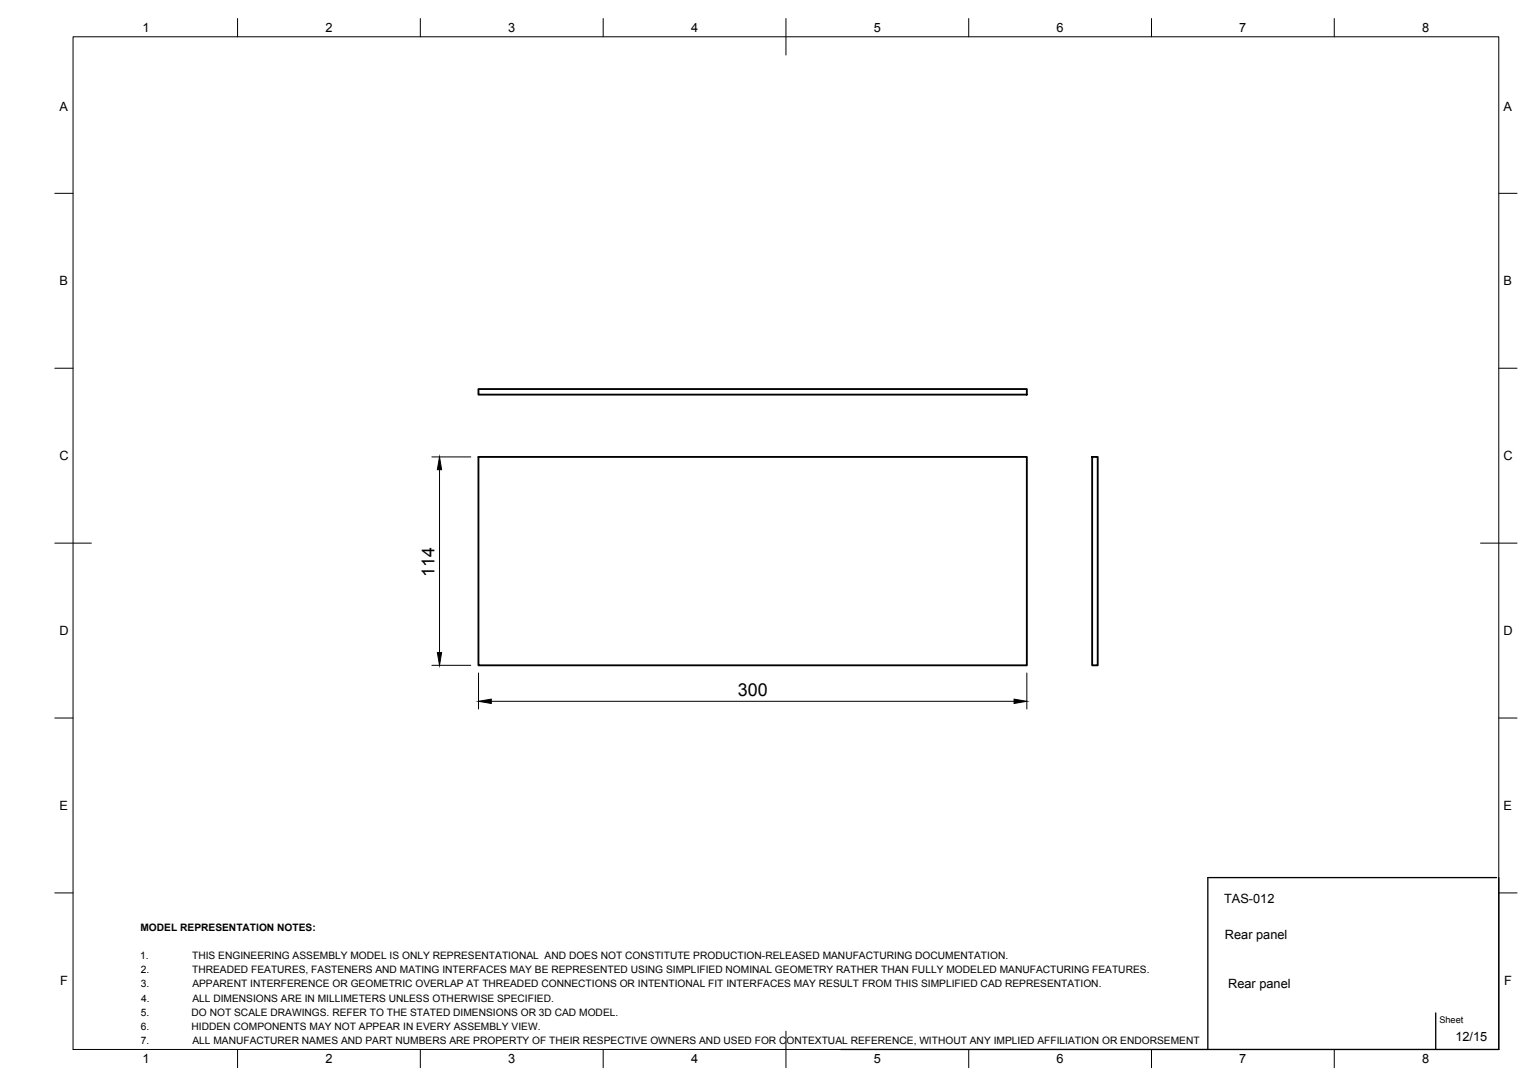
ISO-10303-21;
HEADER;
/* Generated by software containing ST-Developer
 * from STEP Tools, Inc. (www.steptools.com) 
 */

FILE_DESCRIPTION(
/* description */ (
'Independent welded steel electronics enclosure with removable sealed 
lid, internal mounting tray and two threaded cable entries. 300 x 220 
mm body. No ingress or electrical safety rating assigned.'),
/* implementation_level */ '2;1');

FILE_NAME(
/* name */ 'Rear panel.step',
/* time_stamp */ '2026-11-14T09:13:27-08:00',
/* author */ (''),
/* organization */ (''),
/* preprocessor_version */ 'ST-DEVELOPER v20.2',
/* originating_system */ 'Autodesk Translation Framework v15.17.0.0',
/* authorisation */ '');

FILE_SCHEMA (('AUTOMOTIVE_DESIGN { 1 0 10303 214 3 1 1 }'));
ENDSEC;

DATA;
#10=MECHANICAL_DESIGN_GEOMETRIC_PRESENTATION_REPRESENTATION('',(#968),#94412);
#938=SHAPE_REPRESENTATION_RELATIONSHIP('SRR','None',#94490,#953);
#953=ADVANCED_BREP_SHAPE_REPRESENTATION('',(#983),#94399);
#968=STYLED_ITEM('',(#94576),#983);
#983=MANIFOLD_SOLID_BREP('Body1',#8253);
#1070=PLANE('',#8467);
#1071=PLANE('',#8468);
#1072=PLANE('',#8469);
#1073=PLANE('',#8470);
#1074=PLANE('',#8471);
#1075=PLANE('',#8472);
#1176=FACE_OUTER_BOUND('',#1544,.T.);
#1177=FACE_OUTER_BOUND('',#1545,.T.);
#1178=FACE_OUTER_BOUND('',#1546,.T.);
#1179=FACE_OUTER_BOUND('',#1547,.T.);
#1180=FACE_OUTER_BOUND('',#1548,.T.);
#1181=FACE_OUTER_BOUND('',#1549,.T.);
#1544=EDGE_LOOP('',(#5178,#5179,#5180,#5181));
#1545=EDGE_LOOP('',(#5182,#5183,#5184,#5185));
#1546=EDGE_LOOP('',(#5186,#5187,#5188,#5189));
#1547=EDGE_LOOP('',(#5190,#5191,#5192,#5193));
#1548=EDGE_LOOP('',(#5194,#5195,#5196,#5197));
#1549=EDGE_LOOP('',(#5198,#5199,#5200,#5201));
#1962=LINE('',#10456,#2360);
#1963=LINE('',#10458,#2361);
#1964=LINE('',#10460,#2362);
#1965=LINE('',#10461,#2363);
#1966=LINE('',#10464,#2364);
#1967=LINE('',#10466,#2365);
#1968=LINE('',#10467,#2366);
#1969=LINE('',#10470,#2367);
#1970=LINE('',#10472,#2368);
#1971=LINE('',#10473,#2369);
#1972=LINE('',#10475,#2370);
#1973=LINE('',#10476,#2371);
#2360=VECTOR('',#9044,10.);
#2361=VECTOR('',#9045,10.);
#2362=VECTOR('',#9046,10.);
#2363=VECTOR('',#9047,10.);
#2364=VECTOR('',#9050,10.);
#2365=VECTOR('',#9051,10.);
#2366=VECTOR('',#9052,10.);
#2367=VECTOR('',#9055,10.);
#2368=VECTOR('',#9056,10.);
#2369=VECTOR('',#9057,10.);
#2370=VECTOR('',#9060,10.);
#2371=VECTOR('',#9061,10.);
#2874=VERTEX_POINT('',#10454);
#2875=VERTEX_POINT('',#10455);
#2876=VERTEX_POINT('',#10457);
#2877=VERTEX_POINT('',#10459);
#2878=VERTEX_POINT('',#10463);
#2879=VERTEX_POINT('',#10465);
#2880=VERTEX_POINT('',#10469);
#2881=VERTEX_POINT('',#10471);
#3854=EDGE_CURVE('',#2874,#2875,#1962,.T.);
#3855=EDGE_CURVE('',#2875,#2876,#1963,.T.);
#3856=EDGE_CURVE('',#2877,#2876,#1964,.T.);
#3857=EDGE_CURVE('',#2874,#2877,#1965,.T.);
#3858=EDGE_CURVE('',#2878,#2874,#1966,.T.);
#3859=EDGE_CURVE('',#2879,#2877,#1967,.T.);
#3860=EDGE_CURVE('',#2878,#2879,#1968,.T.);
#3861=EDGE_CURVE('',#2880,#2878,#1969,.T.);
#3862=EDGE_CURVE('',#2881,#2879,#1970,.T.);
#3863=EDGE_CURVE('',#2880,#2881,#1971,.T.);
#3864=EDGE_CURVE('',#2875,#2880,#1972,.T.);
#3865=EDGE_CURVE('',#2876,#2881,#1973,.T.);
#5178=ORIENTED_EDGE('',*,*,#3854,.T.);
#5179=ORIENTED_EDGE('',*,*,#3855,.T.);
#5180=ORIENTED_EDGE('',*,*,#3856,.F.);
#5181=ORIENTED_EDGE('',*,*,#3857,.F.);
#5182=ORIENTED_EDGE('',*,*,#3858,.T.);
#5183=ORIENTED_EDGE('',*,*,#3857,.T.);
#5184=ORIENTED_EDGE('',*,*,#3859,.F.);
#5185=ORIENTED_EDGE('',*,*,#3860,.F.);
#5186=ORIENTED_EDGE('',*,*,#3861,.T.);
#5187=ORIENTED_EDGE('',*,*,#3860,.T.);
#5188=ORIENTED_EDGE('',*,*,#3862,.F.);
#5189=ORIENTED_EDGE('',*,*,#3863,.F.);
#5190=ORIENTED_EDGE('',*,*,#3864,.T.);
#5191=ORIENTED_EDGE('',*,*,#3863,.T.);
#5192=ORIENTED_EDGE('',*,*,#3865,.F.);
#5193=ORIENTED_EDGE('',*,*,#3855,.F.);
#5194=ORIENTED_EDGE('',*,*,#3865,.T.);
#5195=ORIENTED_EDGE('',*,*,#3862,.T.);
#5196=ORIENTED_EDGE('',*,*,#3859,.T.);
#5197=ORIENTED_EDGE('',*,*,#3856,.T.);
#5198=ORIENTED_EDGE('',*,*,#3864,.F.);
#5199=ORIENTED_EDGE('',*,*,#3854,.F.);
#5200=ORIENTED_EDGE('',*,*,#3858,.F.);
#5201=ORIENTED_EDGE('',*,*,#3861,.F.);
#7913=ADVANCED_FACE('',(#1176),#1070,.T.);
#7914=ADVANCED_FACE('',(#1177),#1071,.T.);
#7915=ADVANCED_FACE('',(#1178),#1072,.T.);
#7916=ADVANCED_FACE('',(#1179),#1073,.T.);
#7917=ADVANCED_FACE('',(#1180),#1074,.T.);
#7918=ADVANCED_FACE('',(#1181),#1075,.F.);
#8253=CLOSED_SHELL('',(#7913,#7914,#7915,#7916,#7917,#7918));
#8466=AXIS2_PLACEMENT_3D('',#10452,#9040,#9041);
#8467=AXIS2_PLACEMENT_3D('',#10453,#9042,#9043);
#8468=AXIS2_PLACEMENT_3D('',#10462,#9048,#9049);
#8469=AXIS2_PLACEMENT_3D('',#10468,#9053,#9054);
#8470=AXIS2_PLACEMENT_3D('',#10474,#9058,#9059);
#8471=AXIS2_PLACEMENT_3D('',#10477,#9062,#9063);
#8472=AXIS2_PLACEMENT_3D('',#10478,#9064,#9065);
#9040=DIRECTION('axis',(0.,0.,1.));
#9041=DIRECTION('refdir',(1.,0.,0.));
#9042=DIRECTION('center_axis',(0.,1.,0.));
#9043=DIRECTION('ref_axis',(-1.,0.,0.));
#9044=DIRECTION('',(-1.,0.,0.));
#9045=DIRECTION('',(0.,0.,1.));
#9046=DIRECTION('',(-1.,0.,0.));
#9047=DIRECTION('',(0.,0.,1.));
#9048=DIRECTION('center_axis',(1.,0.,0.));
#9049=DIRECTION('ref_axis',(0.,1.,0.));
#9050=DIRECTION('',(0.,1.,0.));
#9051=DIRECTION('',(0.,1.,0.));
#9052=DIRECTION('',(0.,0.,1.));
#9053=DIRECTION('center_axis',(0.,-1.,0.));
#9054=DIRECTION('ref_axis',(1.,0.,0.));
#9055=DIRECTION('',(1.,0.,0.));
#9056=DIRECTION('',(1.,0.,0.));
#9057=DIRECTION('',(0.,0.,1.));
#9058=DIRECTION('center_axis',(-1.,0.,0.));
#9059=DIRECTION('ref_axis',(0.,-1.,0.));
#9060=DIRECTION('',(0.,-1.,0.));
#9061=DIRECTION('',(0.,-1.,0.));
#9062=DIRECTION('center_axis',(0.,0.,1.));
#9063=DIRECTION('ref_axis',(1.,0.,0.));
#9064=DIRECTION('center_axis',(0.,0.,1.));
#9065=DIRECTION('ref_axis',(1.,0.,0.));
#10452=CARTESIAN_POINT('',(0.,0.,0.));
#10453=CARTESIAN_POINT('Origin',(150.,1.5,0.));
#10454=CARTESIAN_POINT('',(150.,1.5,0.));
#10455=CARTESIAN_POINT('',(-150.,1.5,0.));
#10456=CARTESIAN_POINT('',(150.,1.5,0.));
#10457=CARTESIAN_POINT('',(-150.,1.5,114.));
#10458=CARTESIAN_POINT('',(-150.,1.5,0.));
#10459=CARTESIAN_POINT('',(150.,1.5,114.));
#10460=CARTESIAN_POINT('',(150.,1.5,114.));
#10461=CARTESIAN_POINT('',(150.,1.5,0.));
#10462=CARTESIAN_POINT('Origin',(150.,-1.5,0.));
#10463=CARTESIAN_POINT('',(150.,-1.5,0.));
#10464=CARTESIAN_POINT('',(150.,-1.5,0.));
#10465=CARTESIAN_POINT('',(150.,-1.5,114.));
#10466=CARTESIAN_POINT('',(150.,-1.5,114.));
#10467=CARTESIAN_POINT('',(150.,-1.5,0.));
#10468=CARTESIAN_POINT('Origin',(-150.,-1.5,0.));
#10469=CARTESIAN_POINT('',(-150.,-1.5,0.));
#10470=CARTESIAN_POINT('',(-150.,-1.5,0.));
#10471=CARTESIAN_POINT('',(-150.,-1.5,114.));
#10472=CARTESIAN_POINT('',(-150.,-1.5,114.));
#10473=CARTESIAN_POINT('',(-150.,-1.5,0.));
#10474=CARTESIAN_POINT('Origin',(-150.,1.5,0.));
#10475=CARTESIAN_POINT('',(-150.,1.5,0.));
#10476=CARTESIAN_POINT('',(-150.,1.5,114.));
#10477=CARTESIAN_POINT('Origin',(0.,0.,114.));
#10478=CARTESIAN_POINT('Origin',(0.,0.,0.));
#94381=UNCERTAINTY_MEASURE_WITH_UNIT(LENGTH_MEASURE(0.01),#94413,
'DISTANCE_ACCURACY_VALUE',
'Maximum model space distance between geometric entities at asserted c
onnectivities');
#94394=UNCERTAINTY_MEASURE_WITH_UNIT(LENGTH_MEASURE(0.01),#94413,
'DISTANCE_ACCURACY_VALUE',
'Maximum model space distance between geometric entities at asserted c
onnectivities');
#94399=(
GEOMETRIC_REPRESENTATION_CONTEXT(3)
GLOBAL_UNCERTAINTY_ASSIGNED_CONTEXT((#94381))
GLOBAL_UNIT_ASSIGNED_CONTEXT((#94413,#94415,#94416))
REPRESENTATION_CONTEXT('','3D')
);
#94412=(
GEOMETRIC_REPRESENTATION_CONTEXT(3)
GLOBAL_UNCERTAINTY_ASSIGNED_CONTEXT((#94394))
GLOBAL_UNIT_ASSIGNED_CONTEXT((#94413,#94415,#94416))
REPRESENTATION_CONTEXT('','3D')
);
#94413=(
LENGTH_UNIT()
NAMED_UNIT(*)
SI_UNIT(.MILLI.,.METRE.)
);
#94415=(
NAMED_UNIT(*)
PLANE_ANGLE_UNIT()
SI_UNIT($,.RADIAN.)
);
#94416=(
NAMED_UNIT(*)
SI_UNIT($,.STERADIAN.)
SOLID_ANGLE_UNIT()
);
#94421=SHAPE_DEFINITION_REPRESENTATION(#94438,#94490);
#94438=PRODUCT_DEFINITION_SHAPE('',$,#94508);
#94490=SHAPE_REPRESENTATION('',(#8466),#94399);
#94503=PRODUCT_DEFINITION_CONTEXT('part definition',#94556,'design');
#94508=PRODUCT_DEFINITION('Rear panel','Rear panel',#94525,#94503);
#94525=PRODUCT_DEFINITION_FORMATION('',$,#94562);
#94556=APPLICATION_CONTEXT(
'Core Data for Automotive Mechanical Design Process');
#94557=PRODUCT_CONTEXT('part definition',#94556,'mechanical');
#94562=PRODUCT('Rear panel','Rear panel',
'3 mm steel sheet; weld adjoining shell-panel edges continuously. Fabr
ication weld specification remains to be selected.',(#94557));
#94576=PRESENTATION_STYLE_ASSIGNMENT((#94583));
#94583=SURFACE_STYLE_USAGE(.BOTH.,#94590);
#94590=SURFACE_SIDE_STYLE('',(#94597));
#94597=SURFACE_STYLE_FILL_AREA(#94604);
#94604=FILL_AREA_STYLE('Opaque(23,69,131)',(#94611));
#94611=FILL_AREA_STYLE_COLOUR('Opaque(23,69,131)',#94618);
#94618=COLOUR_RGB('Opaque(23,69,131)',0.0901960784313725,0.270588235294118,
0.513725490196078);
ENDSEC;
END-ISO-10303-21;
